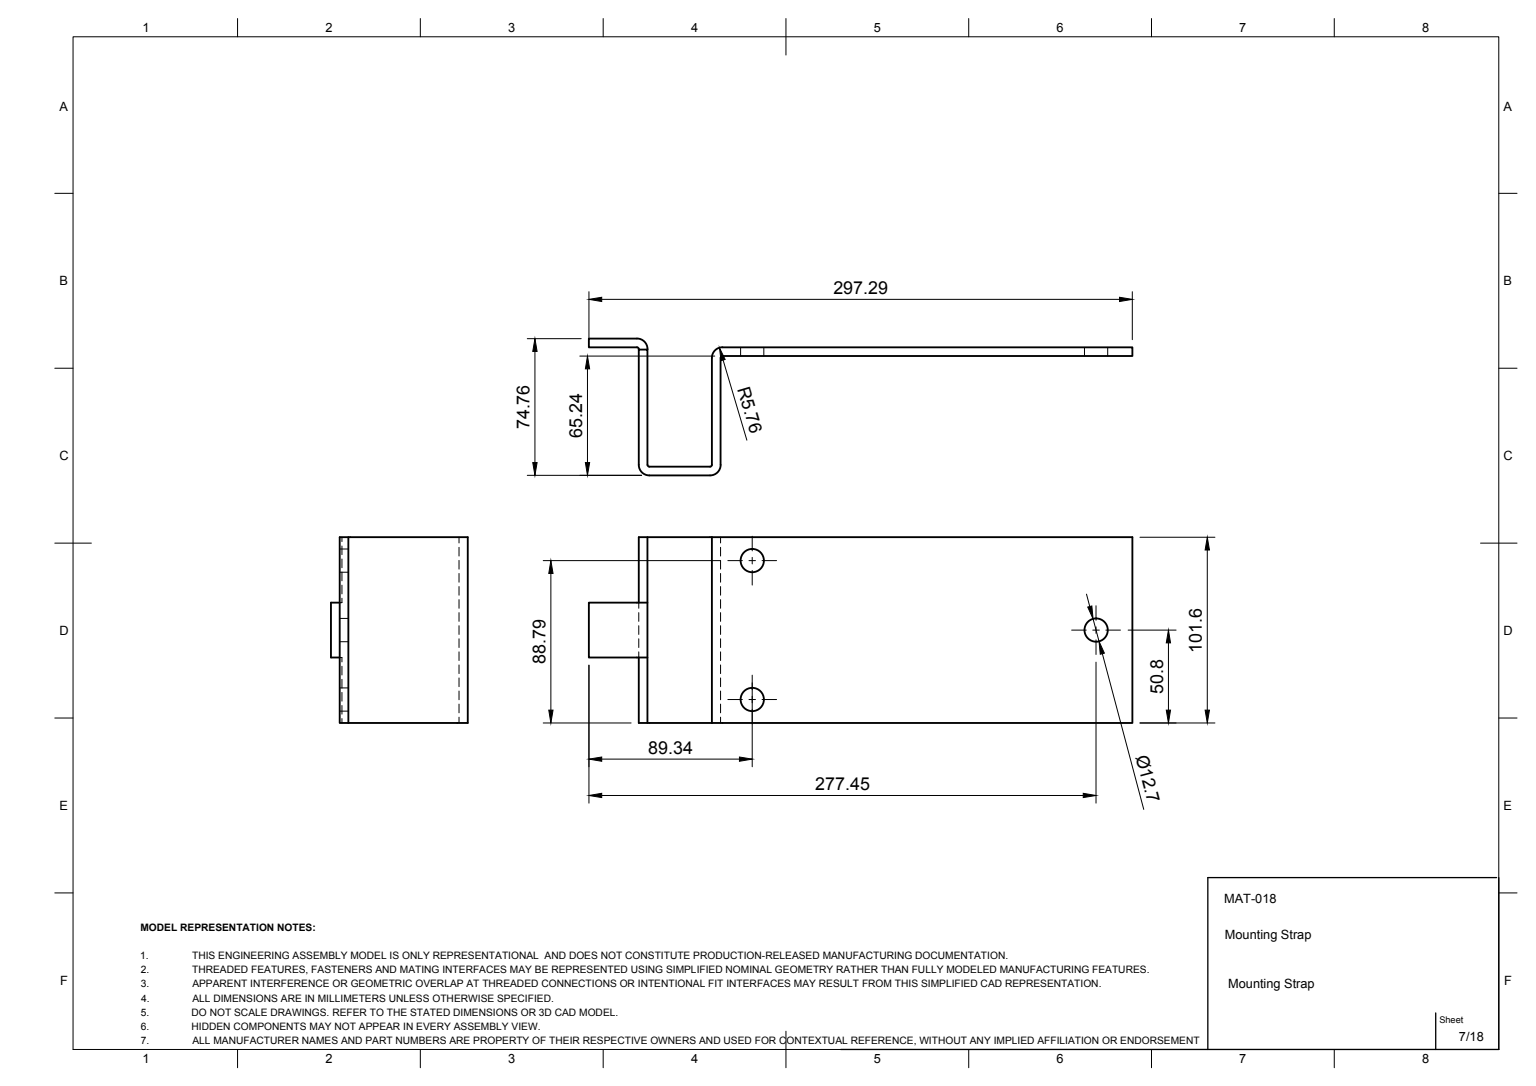
ISO-10303-21;
HEADER;
/* Generated by software containing ST-Developer
 * from STEP Tools, Inc. (www.steptools.com) 
 */

FILE_DESCRIPTION(
/* description */ ('STEP AP214'),
/* implementation_level */ '2;1');

FILE_NAME(
/* name */ 'Mounting Strap.step',
/* time_stamp */ '2026-11-14T06:16:09-08:00',
/* author */ (''),
/* organization */ (''),
/* preprocessor_version */ 'ST-DEVELOPER v20.2',
/* originating_system */ 'Autodesk Translation Framework v15.17.0.0',
/* authorisation */ '');

FILE_SCHEMA (('AUTOMOTIVE_DESIGN { 1 0 10303 214 3 1 1 }'));
ENDSEC;

DATA;
#10=MECHANICAL_DESIGN_GEOMETRIC_PRESENTATION_REPRESENTATION('',(#351),#18006);
#319=SHAPE_REPRESENTATION_RELATIONSHIP('SRR','None',#18075,#335);
#335=ADVANCED_BREP_SHAPE_REPRESENTATION('',(#367),#17992);
#351=STYLED_ITEM('',(#18172),#367);
#367=MANIFOLD_SOLID_BREP('Body1',#9560);
#449=FACE_BOUND('',#1749,.T.);
#450=FACE_BOUND('',#1750,.T.);
#451=FACE_BOUND('',#1751,.T.);
#452=FACE_BOUND('',#1754,.T.);
#453=FACE_BOUND('',#1755,.T.);
#454=FACE_BOUND('',#1756,.T.);
#662=PLANE('',#10157);
#663=PLANE('',#10160);
#664=PLANE('',#10161);
#665=PLANE('',#10164);
#666=PLANE('',#10165);
#667=PLANE('',#10168);
#668=PLANE('',#10169);
#669=PLANE('',#10172);
#670=PLANE('',#10173);
#671=PLANE('',#10176);
#672=PLANE('',#10177);
#673=PLANE('',#10180);
#674=PLANE('',#10181);
#675=PLANE('',#10182);
#676=PLANE('',#10183);
#677=PLANE('',#10184);
#678=PLANE('',#10188);
#679=PLANE('',#10190);
#680=PLANE('',#10192);
#681=PLANE('',#10194);
#682=PLANE('',#10195);
#683=PLANE('',#10196);
#684=PLANE('',#10198);
#685=PLANE('',#10200);
#686=PLANE('',#10202);
#687=PLANE('',#10206);
#688=PLANE('',#10207);
#689=PLANE('',#10208);
#690=PLANE('',#10209);
#691=PLANE('',#10210);
#1076=FACE_OUTER_BOUND('',#1722,.T.);
#1077=FACE_OUTER_BOUND('',#1723,.T.);
#1078=FACE_OUTER_BOUND('',#1724,.T.);
#1079=FACE_OUTER_BOUND('',#1725,.T.);
#1080=FACE_OUTER_BOUND('',#1726,.T.);
#1081=FACE_OUTER_BOUND('',#1727,.T.);
#1082=FACE_OUTER_BOUND('',#1728,.T.);
#1083=FACE_OUTER_BOUND('',#1729,.T.);
#1084=FACE_OUTER_BOUND('',#1730,.T.);
#1085=FACE_OUTER_BOUND('',#1731,.T.);
#1086=FACE_OUTER_BOUND('',#1732,.T.);
#1087=FACE_OUTER_BOUND('',#1733,.T.);
#1088=FACE_OUTER_BOUND('',#1734,.T.);
#1089=FACE_OUTER_BOUND('',#1735,.T.);
#1090=FACE_OUTER_BOUND('',#1736,.T.);
#1091=FACE_OUTER_BOUND('',#1737,.T.);
#1092=FACE_OUTER_BOUND('',#1738,.T.);
#1093=FACE_OUTER_BOUND('',#1739,.T.);
#1094=FACE_OUTER_BOUND('',#1740,.T.);
#1095=FACE_OUTER_BOUND('',#1741,.T.);
#1096=FACE_OUTER_BOUND('',#1742,.T.);
#1097=FACE_OUTER_BOUND('',#1743,.T.);
#1098=FACE_OUTER_BOUND('',#1744,.T.);
#1099=FACE_OUTER_BOUND('',#1745,.T.);
#1100=FACE_OUTER_BOUND('',#1746,.T.);
#1101=FACE_OUTER_BOUND('',#1747,.T.);
#1102=FACE_OUTER_BOUND('',#1748,.T.);
#1103=FACE_OUTER_BOUND('',#1752,.T.);
#1104=FACE_OUTER_BOUND('',#1753,.T.);
#1105=FACE_OUTER_BOUND('',#1757,.T.);
#1106=FACE_OUTER_BOUND('',#1758,.T.);
#1107=FACE_OUTER_BOUND('',#1759,.T.);
#1108=FACE_OUTER_BOUND('',#1760,.T.);
#1109=FACE_OUTER_BOUND('',#1761,.T.);
#1110=FACE_OUTER_BOUND('',#1762,.T.);
#1111=FACE_OUTER_BOUND('',#1763,.T.);
#1112=FACE_OUTER_BOUND('',#1764,.T.);
#1113=FACE_OUTER_BOUND('',#1765,.T.);
#1114=FACE_OUTER_BOUND('',#1766,.T.);
#1115=FACE_OUTER_BOUND('',#1767,.T.);
#1116=FACE_OUTER_BOUND('',#1768,.T.);
#1722=EDGE_LOOP('',(#7242,#7243,#7244,#7245));
#1723=EDGE_LOOP('',(#7246,#7247,#7248,#7249));
#1724=EDGE_LOOP('',(#7250,#7251,#7252,#7253));
#1725=EDGE_LOOP('',(#7254,#7255,#7256,#7257));
#1726=EDGE_LOOP('',(#7258,#7259,#7260,#7261));
#1727=EDGE_LOOP('',(#7262,#7263,#7264,#7265));
#1728=EDGE_LOOP('',(#7266,#7267,#7268,#7269));
#1729=EDGE_LOOP('',(#7270,#7271,#7272,#7273));
#1730=EDGE_LOOP('',(#7274,#7275,#7276,#7277));
#1731=EDGE_LOOP('',(#7278,#7279,#7280,#7281));
#1732=EDGE_LOOP('',(#7282,#7283,#7284,#7285));
#1733=EDGE_LOOP('',(#7286,#7287,#7288,#7289));
#1734=EDGE_LOOP('',(#7290,#7291,#7292,#7293));
#1735=EDGE_LOOP('',(#7294,#7295,#7296,#7297));
#1736=EDGE_LOOP('',(#7298,#7299,#7300,#7301));
#1737=EDGE_LOOP('',(#7302,#7303,#7304,#7305));
#1738=EDGE_LOOP('',(#7306,#7307,#7308,#7309));
#1739=EDGE_LOOP('',(#7310,#7311,#7312,#7313));
#1740=EDGE_LOOP('',(#7314,#7315,#7316,#7317));
#1741=EDGE_LOOP('',(#7318,#7319,#7320,#7321));
#1742=EDGE_LOOP('',(#7322,#7323,#7324,#7325,#7326,#7327,#7328,#7329));
#1743=EDGE_LOOP('',(#7330,#7331,#7332,#7333));
#1744=EDGE_LOOP('',(#7334,#7335,#7336,#7337));
#1745=EDGE_LOOP('',(#7338,#7339,#7340,#7341));
#1746=EDGE_LOOP('',(#7342,#7343,#7344,#7345));
#1747=EDGE_LOOP('',(#7346,#7347,#7348,#7349));
#1748=EDGE_LOOP('',(#7350,#7351,#7352,#7353));
#1749=EDGE_LOOP('',(#7354));
#1750=EDGE_LOOP('',(#7355));
#1751=EDGE_LOOP('',(#7356));
#1752=EDGE_LOOP('',(#7357,#7358,#7359,#7360));
#1753=EDGE_LOOP('',(#7361,#7362,#7363,#7364));
#1754=EDGE_LOOP('',(#7365));
#1755=EDGE_LOOP('',(#7366));
#1756=EDGE_LOOP('',(#7367));
#1757=EDGE_LOOP('',(#7368,#7369,#7370,#7371));
#1758=EDGE_LOOP('',(#7372,#7373,#7374,#7375));
#1759=EDGE_LOOP('',(#7376,#7377,#7378,#7379));
#1760=EDGE_LOOP('',(#7380,#7381,#7382,#7383));
#1761=EDGE_LOOP('',(#7384,#7385,#7386,#7387));
#1762=EDGE_LOOP('',(#7388,#7389,#7390,#7391,#7392,#7393,#7394,#7395));
#1763=EDGE_LOOP('',(#7396,#7397,#7398,#7399));
#1764=EDGE_LOOP('',(#7400,#7401,#7402,#7403));
#1765=EDGE_LOOP('',(#7404,#7405,#7406,#7407,#7408,#7409,#7410,#7411));
#1766=EDGE_LOOP('',(#7412,#7413,#7414,#7415));
#1767=EDGE_LOOP('',(#7416,#7417,#7418,#7419,#7420,#7421,#7422,#7423));
#1768=EDGE_LOOP('',(#7424,#7425,#7426,#7427));
#2503=LINE('',#14917,#3227);
#2504=LINE('',#14923,#3228);
#2505=LINE('',#14929,#3229);
#2506=LINE('',#14934,#3230);
#2507=LINE('',#14938,#3231);
#2508=LINE('',#14942,#3232);
#2509=LINE('',#14944,#3233);
#2510=LINE('',#14945,#3234);
#2511=LINE('',#14949,#3235);
#2512=LINE('',#14953,#3236);
#2513=LINE('',#14957,#3237);
#2514=LINE('',#14959,#3238);
#2515=LINE('',#14960,#3239);
#2516=LINE('',#14964,#3240);
#2517=LINE('',#14969,#3241);
#2518=LINE('',#14971,#3242);
#2519=LINE('',#14972,#3243);
#2520=LINE('',#14976,#3244);
#2521=LINE('',#14980,#3245);
#2522=LINE('',#14983,#3246);
#2523=LINE('',#14984,#3247);
#2524=LINE('',#14988,#3248);
#2525=LINE('',#14994,#3249);
#2526=LINE('',#14995,#3250);
#2527=LINE('',#14996,#3251);
#2528=LINE('',#15000,#3252);
#2529=LINE('',#15004,#3253);
#2530=LINE('',#15007,#3254);
#2531=LINE('',#15008,#3255);
#2532=LINE('',#15012,#3256);
#2533=LINE('',#15013,#3257);
#2534=LINE('',#15014,#3258);
#2535=LINE('',#15018,#3259);
#2536=LINE('',#15020,#3260);
#2537=LINE('',#15022,#3261);
#2538=LINE('',#15023,#3262);
#2539=LINE('',#15026,#3263);
#2540=LINE('',#15028,#3264);
#2541=LINE('',#15029,#3265);
#2542=LINE('',#15032,#3266);
#2543=LINE('',#15034,#3267);
#2544=LINE('',#15035,#3268);
#2545=LINE('',#15041,#3269);
#2546=LINE('',#15044,#3270);
#2547=LINE('',#15046,#3271);
#2548=LINE('',#15047,#3272);
#2549=LINE('',#15048,#3273);
#2550=LINE('',#15049,#3274);
#2551=LINE('',#15051,#3275);
#2552=LINE('',#15053,#3276);
#2553=LINE('',#15055,#3277);
#2554=LINE('',#15057,#3278);
#2555=LINE('',#15059,#3279);
#2556=LINE('',#15062,#3280);
#2557=LINE('',#15063,#3281);
#2558=LINE('',#15066,#3282);
#2559=LINE('',#15067,#3283);
#2560=LINE('',#15069,#3284);
#2561=LINE('',#15070,#3285);
#2562=LINE('',#15072,#3286);
#2563=LINE('',#15074,#3287);
#2564=LINE('',#15076,#3288);
#2565=LINE('',#15078,#3289);
#2566=LINE('',#15080,#3290);
#2567=LINE('',#15084,#3291);
#2568=LINE('',#15086,#3292);
#2569=LINE('',#15087,#3293);
#2570=LINE('',#15089,#3294);
#2571=LINE('',#15090,#3295);
#2572=LINE('',#15096,#3296);
#2573=LINE('',#15099,#3297);
#3227=VECTOR('',#12050,6.34999999999999);
#3228=VECTOR('',#12057,6.34999999999999);
#3229=VECTOR('',#12064,6.35);
#3230=VECTOR('',#12069,1000.);
#3231=VECTOR('',#12072,1000.);
#3232=VECTOR('',#12077,1000.);
#3233=VECTOR('',#12078,1000.);
#3234=VECTOR('',#12079,1000.);
#3235=VECTOR('',#12082,1000.);
#3236=VECTOR('',#12085,1000.);
#3237=VECTOR('',#12090,1000.);
#3238=VECTOR('',#12091,1000.);
#3239=VECTOR('',#12092,1000.);
#3240=VECTOR('',#12095,1000.);
#3241=VECTOR('',#12102,1000.);
#3242=VECTOR('',#12103,1000.);
#3243=VECTOR('',#12104,1000.);
#3244=VECTOR('',#12107,1000.);
#3245=VECTOR('',#12110,1000.);
#3246=VECTOR('',#12115,1000.);
#3247=VECTOR('',#12116,1000.);
#3248=VECTOR('',#12119,1000.);
#3249=VECTOR('',#12126,1000.);
#3250=VECTOR('',#12127,1000.);
#3251=VECTOR('',#12128,1000.);
#3252=VECTOR('',#12131,1000.);
#3253=VECTOR('',#12134,1000.);
#3254=VECTOR('',#12139,1000.);
#3255=VECTOR('',#12140,1000.);
#3256=VECTOR('',#12143,1000.);
#3257=VECTOR('',#12144,1000.);
#3258=VECTOR('',#12145,1000.);
#3259=VECTOR('',#12148,1000.);
#3260=VECTOR('',#12149,1000.);
#3261=VECTOR('',#12150,1000.);
#3262=VECTOR('',#12151,1000.);
#3263=VECTOR('',#12154,1000.);
#3264=VECTOR('',#12155,1000.);
#3265=VECTOR('',#12156,1000.);
#3266=VECTOR('',#12159,1000.);
#3267=VECTOR('',#12160,1000.);
#3268=VECTOR('',#12161,1000.);
#3269=VECTOR('',#12168,1000.);
#3270=VECTOR('',#12171,1000.);
#3271=VECTOR('',#12172,1000.);
#3272=VECTOR('',#12173,1000.);
#3273=VECTOR('',#12174,1000.);
#3274=VECTOR('',#12175,1000.);
#3275=VECTOR('',#12178,1000.);
#3276=VECTOR('',#12181,1000.);
#3277=VECTOR('',#12184,1000.);
#3278=VECTOR('',#12187,1000.);
#3279=VECTOR('',#12190,1000.);
#3280=VECTOR('',#12193,1000.);
#3281=VECTOR('',#12194,1000.);
#3282=VECTOR('',#12197,1000.);
#3283=VECTOR('',#12198,1000.);
#3284=VECTOR('',#12201,1000.);
#3285=VECTOR('',#12202,1000.);
#3286=VECTOR('',#12205,1000.);
#3287=VECTOR('',#12208,1000.);
#3288=VECTOR('',#12211,1000.);
#3289=VECTOR('',#12214,1000.);
#3290=VECTOR('',#12217,1000.);
#3291=VECTOR('',#12220,1000.);
#3292=VECTOR('',#12221,1000.);
#3293=VECTOR('',#12222,1000.);
#3294=VECTOR('',#12223,1000.);
#3295=VECTOR('',#12224,1000.);
#3296=VECTOR('',#12235,1000.);
#3297=VECTOR('',#12240,1000.);
#3714=CIRCLE('',#10149,6.34999999999999);
#3715=CIRCLE('',#10150,6.34999999999999);
#3716=CIRCLE('',#10152,6.34999999999999);
#3717=CIRCLE('',#10153,6.34999999999999);
#3718=CIRCLE('',#10155,6.35);
#3719=CIRCLE('',#10156,6.35);
#3720=CIRCLE('',#10158,1.);
#3721=CIRCLE('',#10159,5.7625);
#3722=CIRCLE('',#10162,1.);
#3723=CIRCLE('',#10163,5.7625);
#3724=CIRCLE('',#10166,5.7625);
#3725=CIRCLE('',#10167,1.);
#3726=CIRCLE('',#10170,5.7625);
#3727=CIRCLE('',#10171,1.);
#3728=CIRCLE('',#10174,5.7625);
#3729=CIRCLE('',#10175,1.);
#3730=CIRCLE('',#10178,5.7625);
#3731=CIRCLE('',#10179,1.);
#3732=CIRCLE('',#10186,1.);
#3733=CIRCLE('',#10187,1.);
#3734=CIRCLE('',#10204,5.7625);
#3735=CIRCLE('',#10205,5.7625);
#4331=VERTEX_POINT('',#14914);
#4332=VERTEX_POINT('',#14916);
#4333=VERTEX_POINT('',#14920);
#4334=VERTEX_POINT('',#14922);
#4335=VERTEX_POINT('',#14926);
#4336=VERTEX_POINT('',#14928);
#4337=VERTEX_POINT('',#14932);
#4338=VERTEX_POINT('',#14933);
#4339=VERTEX_POINT('',#14935);
#4340=VERTEX_POINT('',#14937);
#4341=VERTEX_POINT('',#14941);
#4342=VERTEX_POINT('',#14943);
#4343=VERTEX_POINT('',#14947);
#4344=VERTEX_POINT('',#14948);
#4345=VERTEX_POINT('',#14950);
#4346=VERTEX_POINT('',#14952);
#4347=VERTEX_POINT('',#14956);
#4348=VERTEX_POINT('',#14958);
#4349=VERTEX_POINT('',#14962);
#4350=VERTEX_POINT('',#14963);
#4351=VERTEX_POINT('',#14968);
#4352=VERTEX_POINT('',#14970);
#4353=VERTEX_POINT('',#14974);
#4354=VERTEX_POINT('',#14975);
#4355=VERTEX_POINT('',#14977);
#4356=VERTEX_POINT('',#14979);
#4357=VERTEX_POINT('',#14986);
#4358=VERTEX_POINT('',#14987);
#4359=VERTEX_POINT('',#14992);
#4360=VERTEX_POINT('',#14993);
#4361=VERTEX_POINT('',#14998);
#4362=VERTEX_POINT('',#14999);
#4363=VERTEX_POINT('',#15001);
#4364=VERTEX_POINT('',#15003);
#4365=VERTEX_POINT('',#15010);
#4366=VERTEX_POINT('',#15011);
#4367=VERTEX_POINT('',#15016);
#4368=VERTEX_POINT('',#15017);
#4369=VERTEX_POINT('',#15019);
#4370=VERTEX_POINT('',#15021);
#4371=VERTEX_POINT('',#15025);
#4372=VERTEX_POINT('',#15027);
#4373=VERTEX_POINT('',#15031);
#4374=VERTEX_POINT('',#15033);
#4375=VERTEX_POINT('',#15037);
#4376=VERTEX_POINT('',#15039);
#4377=VERTEX_POINT('',#15043);
#4378=VERTEX_POINT('',#15045);
#4379=VERTEX_POINT('',#15061);
#4380=VERTEX_POINT('',#15065);
#4381=VERTEX_POINT('',#15082);
#4382=VERTEX_POINT('',#15083);
#4383=VERTEX_POINT('',#15085);
#4384=VERTEX_POINT('',#15088);
#5369=EDGE_CURVE('',#4331,#4331,#3714,.T.);
#5370=EDGE_CURVE('',#4331,#4332,#2503,.T.);
#5371=EDGE_CURVE('',#4332,#4332,#3715,.T.);
#5372=EDGE_CURVE('',#4333,#4333,#3716,.T.);
#5373=EDGE_CURVE('',#4333,#4334,#2504,.T.);
#5374=EDGE_CURVE('',#4334,#4334,#3717,.T.);
#5375=EDGE_CURVE('',#4335,#4335,#3718,.T.);
#5376=EDGE_CURVE('',#4335,#4336,#2505,.T.);
#5377=EDGE_CURVE('',#4336,#4336,#3719,.T.);
#5378=EDGE_CURVE('',#4337,#4338,#2506,.T.);
#5379=EDGE_CURVE('',#4339,#4337,#3720,.T.);
#5380=EDGE_CURVE('',#4340,#4339,#2507,.T.);
#5381=EDGE_CURVE('',#4340,#4338,#3721,.T.);
#5382=EDGE_CURVE('',#4337,#4341,#2508,.T.);
#5383=EDGE_CURVE('',#4338,#4342,#2509,.T.);
#5384=EDGE_CURVE('',#4342,#4341,#2510,.T.);
#5385=EDGE_CURVE('',#4343,#4344,#2511,.T.);
#5386=EDGE_CURVE('',#4343,#4345,#3722,.T.);
#5387=EDGE_CURVE('',#4346,#4345,#2512,.T.);
#5388=EDGE_CURVE('',#4344,#4346,#3723,.T.);
#5389=EDGE_CURVE('',#4347,#4343,#2513,.T.);
#5390=EDGE_CURVE('',#4348,#4344,#2514,.T.);
#5391=EDGE_CURVE('',#4348,#4347,#2515,.T.);
#5392=EDGE_CURVE('',#4349,#4350,#2516,.T.);
#5393=EDGE_CURVE('',#4341,#4349,#3724,.T.);
#5394=EDGE_CURVE('',#4342,#4350,#3725,.T.);
#5395=EDGE_CURVE('',#4349,#4351,#2517,.T.);
#5396=EDGE_CURVE('',#4350,#4352,#2518,.T.);
#5397=EDGE_CURVE('',#4352,#4351,#2519,.T.);
#5398=EDGE_CURVE('',#4353,#4354,#2520,.T.);
#5399=EDGE_CURVE('',#4353,#4355,#3726,.T.);
#5400=EDGE_CURVE('',#4356,#4355,#2521,.T.);
#5401=EDGE_CURVE('',#4354,#4356,#3727,.T.);
#5402=EDGE_CURVE('',#4345,#4353,#2522,.T.);
#5403=EDGE_CURVE('',#4346,#4354,#2523,.T.);
#5404=EDGE_CURVE('',#4357,#4358,#2524,.T.);
#5405=EDGE_CURVE('',#4351,#4357,#3728,.T.);
#5406=EDGE_CURVE('',#4352,#4358,#3729,.T.);
#5407=EDGE_CURVE('',#4359,#4360,#2525,.T.);
#5408=EDGE_CURVE('',#4357,#4359,#2526,.T.);
#5409=EDGE_CURVE('',#4358,#4360,#2527,.T.);
#5410=EDGE_CURVE('',#4361,#4362,#2528,.T.);
#5411=EDGE_CURVE('',#4361,#4363,#3730,.T.);
#5412=EDGE_CURVE('',#4364,#4363,#2529,.T.);
#5413=EDGE_CURVE('',#4362,#4364,#3731,.T.);
#5414=EDGE_CURVE('',#4355,#4361,#2530,.T.);
#5415=EDGE_CURVE('',#4356,#4362,#2531,.T.);
#5416=EDGE_CURVE('',#4365,#4366,#2532,.T.);
#5417=EDGE_CURVE('',#4364,#4366,#2533,.T.);
#5418=EDGE_CURVE('',#4363,#4365,#2534,.T.);
#5419=EDGE_CURVE('',#4367,#4368,#2535,.T.);
#5420=EDGE_CURVE('',#4367,#4369,#2536,.T.);
#5421=EDGE_CURVE('',#4369,#4370,#2537,.T.);
#5422=EDGE_CURVE('',#4368,#4370,#2538,.T.);
#5423=EDGE_CURVE('',#4367,#4371,#2539,.T.);
#5424=EDGE_CURVE('',#4372,#4368,#2540,.T.);
#5425=EDGE_CURVE('',#4371,#4372,#2541,.T.);
#5426=EDGE_CURVE('',#4371,#4373,#2542,.T.);
#5427=EDGE_CURVE('',#4374,#4372,#2543,.T.);
#5428=EDGE_CURVE('',#4373,#4374,#2544,.T.);
#5429=EDGE_CURVE('',#4373,#4375,#3732,.T.);
#5430=EDGE_CURVE('',#4376,#4374,#3733,.T.);
#5431=EDGE_CURVE('',#4375,#4376,#2545,.T.);
#5432=EDGE_CURVE('',#4375,#4377,#2546,.T.);
#5433=EDGE_CURVE('',#4378,#4376,#2547,.T.);
#5434=EDGE_CURVE('',#4365,#4378,#2548,.T.);
#5435=EDGE_CURVE('',#4357,#4363,#2549,.T.);
#5436=EDGE_CURVE('',#4377,#4359,#2550,.T.);
#5437=EDGE_CURVE('',#4351,#4361,#2551,.T.);
#5438=EDGE_CURVE('',#4349,#4355,#2552,.T.);
#5439=EDGE_CURVE('',#4341,#4353,#2553,.T.);
#5440=EDGE_CURVE('',#4337,#4345,#2554,.T.);
#5441=EDGE_CURVE('',#4339,#4343,#2555,.T.);
#5442=EDGE_CURVE('',#4379,#4347,#2556,.T.);
#5443=EDGE_CURVE('',#4379,#4339,#2557,.T.);
#5444=EDGE_CURVE('',#4380,#4348,#2558,.T.);
#5445=EDGE_CURVE('',#4380,#4379,#2559,.T.);
#5446=EDGE_CURVE('',#4340,#4344,#2560,.T.);
#5447=EDGE_CURVE('',#4380,#4340,#2561,.T.);
#5448=EDGE_CURVE('',#4338,#4346,#2562,.T.);
#5449=EDGE_CURVE('',#4342,#4354,#2563,.T.);
#5450=EDGE_CURVE('',#4350,#4356,#2564,.T.);
#5451=EDGE_CURVE('',#4352,#4362,#2565,.T.);
#5452=EDGE_CURVE('',#4358,#4364,#2566,.T.);
#5453=EDGE_CURVE('',#4381,#4382,#2567,.T.);
#5454=EDGE_CURVE('',#4383,#4381,#2568,.T.);
#5455=EDGE_CURVE('',#4360,#4383,#2569,.T.);
#5456=EDGE_CURVE('',#4384,#4366,#2570,.T.);
#5457=EDGE_CURVE('',#4382,#4384,#2571,.T.);
#5458=EDGE_CURVE('',#4369,#4381,#3734,.T.);
#5459=EDGE_CURVE('',#4382,#4370,#3735,.T.);
#5460=EDGE_CURVE('',#4378,#4384,#2572,.T.);
#5461=EDGE_CURVE('',#4377,#4383,#2573,.T.);
#7242=ORIENTED_EDGE('',*,*,#5369,.F.);
#7243=ORIENTED_EDGE('',*,*,#5370,.T.);
#7244=ORIENTED_EDGE('',*,*,#5371,.T.);
#7245=ORIENTED_EDGE('',*,*,#5370,.F.);
#7246=ORIENTED_EDGE('',*,*,#5372,.F.);
#7247=ORIENTED_EDGE('',*,*,#5373,.T.);
#7248=ORIENTED_EDGE('',*,*,#5374,.T.);
#7249=ORIENTED_EDGE('',*,*,#5373,.F.);
#7250=ORIENTED_EDGE('',*,*,#5375,.F.);
#7251=ORIENTED_EDGE('',*,*,#5376,.T.);
#7252=ORIENTED_EDGE('',*,*,#5377,.T.);
#7253=ORIENTED_EDGE('',*,*,#5376,.F.);
#7254=ORIENTED_EDGE('',*,*,#5378,.F.);
#7255=ORIENTED_EDGE('',*,*,#5379,.F.);
#7256=ORIENTED_EDGE('',*,*,#5380,.F.);
#7257=ORIENTED_EDGE('',*,*,#5381,.T.);
#7258=ORIENTED_EDGE('',*,*,#5382,.F.);
#7259=ORIENTED_EDGE('',*,*,#5378,.T.);
#7260=ORIENTED_EDGE('',*,*,#5383,.T.);
#7261=ORIENTED_EDGE('',*,*,#5384,.T.);
#7262=ORIENTED_EDGE('',*,*,#5385,.F.);
#7263=ORIENTED_EDGE('',*,*,#5386,.T.);
#7264=ORIENTED_EDGE('',*,*,#5387,.F.);
#7265=ORIENTED_EDGE('',*,*,#5388,.F.);
#7266=ORIENTED_EDGE('',*,*,#5389,.T.);
#7267=ORIENTED_EDGE('',*,*,#5385,.T.);
#7268=ORIENTED_EDGE('',*,*,#5390,.F.);
#7269=ORIENTED_EDGE('',*,*,#5391,.T.);
#7270=ORIENTED_EDGE('',*,*,#5392,.F.);
#7271=ORIENTED_EDGE('',*,*,#5393,.F.);
#7272=ORIENTED_EDGE('',*,*,#5384,.F.);
#7273=ORIENTED_EDGE('',*,*,#5394,.T.);
#7274=ORIENTED_EDGE('',*,*,#5395,.F.);
#7275=ORIENTED_EDGE('',*,*,#5392,.T.);
#7276=ORIENTED_EDGE('',*,*,#5396,.T.);
#7277=ORIENTED_EDGE('',*,*,#5397,.T.);
#7278=ORIENTED_EDGE('',*,*,#5398,.F.);
#7279=ORIENTED_EDGE('',*,*,#5399,.T.);
#7280=ORIENTED_EDGE('',*,*,#5400,.F.);
#7281=ORIENTED_EDGE('',*,*,#5401,.F.);
#7282=ORIENTED_EDGE('',*,*,#5402,.T.);
#7283=ORIENTED_EDGE('',*,*,#5398,.T.);
#7284=ORIENTED_EDGE('',*,*,#5403,.F.);
#7285=ORIENTED_EDGE('',*,*,#5387,.T.);
#7286=ORIENTED_EDGE('',*,*,#5404,.F.);
#7287=ORIENTED_EDGE('',*,*,#5405,.F.);
#7288=ORIENTED_EDGE('',*,*,#5397,.F.);
#7289=ORIENTED_EDGE('',*,*,#5406,.T.);
#7290=ORIENTED_EDGE('',*,*,#5407,.F.);
#7291=ORIENTED_EDGE('',*,*,#5408,.F.);
#7292=ORIENTED_EDGE('',*,*,#5404,.T.);
#7293=ORIENTED_EDGE('',*,*,#5409,.T.);
#7294=ORIENTED_EDGE('',*,*,#5410,.F.);
#7295=ORIENTED_EDGE('',*,*,#5411,.T.);
#7296=ORIENTED_EDGE('',*,*,#5412,.F.);
#7297=ORIENTED_EDGE('',*,*,#5413,.F.);
#7298=ORIENTED_EDGE('',*,*,#5414,.T.);
#7299=ORIENTED_EDGE('',*,*,#5410,.T.);
#7300=ORIENTED_EDGE('',*,*,#5415,.F.);
#7301=ORIENTED_EDGE('',*,*,#5400,.T.);
#7302=ORIENTED_EDGE('',*,*,#5416,.T.);
#7303=ORIENTED_EDGE('',*,*,#5417,.F.);
#7304=ORIENTED_EDGE('',*,*,#5412,.T.);
#7305=ORIENTED_EDGE('',*,*,#5418,.T.);
#7306=ORIENTED_EDGE('',*,*,#5419,.F.);
#7307=ORIENTED_EDGE('',*,*,#5420,.T.);
#7308=ORIENTED_EDGE('',*,*,#5421,.T.);
#7309=ORIENTED_EDGE('',*,*,#5422,.F.);
#7310=ORIENTED_EDGE('',*,*,#5423,.F.);
#7311=ORIENTED_EDGE('',*,*,#5419,.T.);
#7312=ORIENTED_EDGE('',*,*,#5424,.F.);
#7313=ORIENTED_EDGE('',*,*,#5425,.F.);
#7314=ORIENTED_EDGE('',*,*,#5426,.F.);
#7315=ORIENTED_EDGE('',*,*,#5425,.T.);
#7316=ORIENTED_EDGE('',*,*,#5427,.F.);
#7317=ORIENTED_EDGE('',*,*,#5428,.F.);
#7318=ORIENTED_EDGE('',*,*,#5429,.F.);
#7319=ORIENTED_EDGE('',*,*,#5428,.T.);
#7320=ORIENTED_EDGE('',*,*,#5430,.F.);
#7321=ORIENTED_EDGE('',*,*,#5431,.F.);
#7322=ORIENTED_EDGE('',*,*,#5432,.F.);
#7323=ORIENTED_EDGE('',*,*,#5431,.T.);
#7324=ORIENTED_EDGE('',*,*,#5433,.F.);
#7325=ORIENTED_EDGE('',*,*,#5434,.F.);
#7326=ORIENTED_EDGE('',*,*,#5418,.F.);
#7327=ORIENTED_EDGE('',*,*,#5435,.F.);
#7328=ORIENTED_EDGE('',*,*,#5408,.T.);
#7329=ORIENTED_EDGE('',*,*,#5436,.F.);
#7330=ORIENTED_EDGE('',*,*,#5411,.F.);
#7331=ORIENTED_EDGE('',*,*,#5437,.F.);
#7332=ORIENTED_EDGE('',*,*,#5405,.T.);
#7333=ORIENTED_EDGE('',*,*,#5435,.T.);
#7334=ORIENTED_EDGE('',*,*,#5414,.F.);
#7335=ORIENTED_EDGE('',*,*,#5438,.F.);
#7336=ORIENTED_EDGE('',*,*,#5395,.T.);
#7337=ORIENTED_EDGE('',*,*,#5437,.T.);
#7338=ORIENTED_EDGE('',*,*,#5399,.F.);
#7339=ORIENTED_EDGE('',*,*,#5439,.F.);
#7340=ORIENTED_EDGE('',*,*,#5393,.T.);
#7341=ORIENTED_EDGE('',*,*,#5438,.T.);
#7342=ORIENTED_EDGE('',*,*,#5402,.F.);
#7343=ORIENTED_EDGE('',*,*,#5440,.F.);
#7344=ORIENTED_EDGE('',*,*,#5382,.T.);
#7345=ORIENTED_EDGE('',*,*,#5439,.T.);
#7346=ORIENTED_EDGE('',*,*,#5386,.F.);
#7347=ORIENTED_EDGE('',*,*,#5441,.F.);
#7348=ORIENTED_EDGE('',*,*,#5379,.T.);
#7349=ORIENTED_EDGE('',*,*,#5440,.T.);
#7350=ORIENTED_EDGE('',*,*,#5389,.F.);
#7351=ORIENTED_EDGE('',*,*,#5442,.F.);
#7352=ORIENTED_EDGE('',*,*,#5443,.T.);
#7353=ORIENTED_EDGE('',*,*,#5441,.T.);
#7354=ORIENTED_EDGE('',*,*,#5371,.F.);
#7355=ORIENTED_EDGE('',*,*,#5374,.F.);
#7356=ORIENTED_EDGE('',*,*,#5377,.F.);
#7357=ORIENTED_EDGE('',*,*,#5391,.F.);
#7358=ORIENTED_EDGE('',*,*,#5444,.F.);
#7359=ORIENTED_EDGE('',*,*,#5445,.T.);
#7360=ORIENTED_EDGE('',*,*,#5442,.T.);
#7361=ORIENTED_EDGE('',*,*,#5390,.T.);
#7362=ORIENTED_EDGE('',*,*,#5446,.F.);
#7363=ORIENTED_EDGE('',*,*,#5447,.F.);
#7364=ORIENTED_EDGE('',*,*,#5444,.T.);
#7365=ORIENTED_EDGE('',*,*,#5369,.T.);
#7366=ORIENTED_EDGE('',*,*,#5372,.T.);
#7367=ORIENTED_EDGE('',*,*,#5375,.T.);
#7368=ORIENTED_EDGE('',*,*,#5388,.T.);
#7369=ORIENTED_EDGE('',*,*,#5448,.F.);
#7370=ORIENTED_EDGE('',*,*,#5381,.F.);
#7371=ORIENTED_EDGE('',*,*,#5446,.T.);
#7372=ORIENTED_EDGE('',*,*,#5403,.T.);
#7373=ORIENTED_EDGE('',*,*,#5449,.F.);
#7374=ORIENTED_EDGE('',*,*,#5383,.F.);
#7375=ORIENTED_EDGE('',*,*,#5448,.T.);
#7376=ORIENTED_EDGE('',*,*,#5401,.T.);
#7377=ORIENTED_EDGE('',*,*,#5450,.F.);
#7378=ORIENTED_EDGE('',*,*,#5394,.F.);
#7379=ORIENTED_EDGE('',*,*,#5449,.T.);
#7380=ORIENTED_EDGE('',*,*,#5415,.T.);
#7381=ORIENTED_EDGE('',*,*,#5451,.F.);
#7382=ORIENTED_EDGE('',*,*,#5396,.F.);
#7383=ORIENTED_EDGE('',*,*,#5450,.T.);
#7384=ORIENTED_EDGE('',*,*,#5413,.T.);
#7385=ORIENTED_EDGE('',*,*,#5452,.F.);
#7386=ORIENTED_EDGE('',*,*,#5406,.F.);
#7387=ORIENTED_EDGE('',*,*,#5451,.T.);
#7388=ORIENTED_EDGE('',*,*,#5453,.F.);
#7389=ORIENTED_EDGE('',*,*,#5454,.F.);
#7390=ORIENTED_EDGE('',*,*,#5455,.F.);
#7391=ORIENTED_EDGE('',*,*,#5409,.F.);
#7392=ORIENTED_EDGE('',*,*,#5452,.T.);
#7393=ORIENTED_EDGE('',*,*,#5417,.T.);
#7394=ORIENTED_EDGE('',*,*,#5456,.F.);
#7395=ORIENTED_EDGE('',*,*,#5457,.F.);
#7396=ORIENTED_EDGE('',*,*,#5421,.F.);
#7397=ORIENTED_EDGE('',*,*,#5458,.T.);
#7398=ORIENTED_EDGE('',*,*,#5453,.T.);
#7399=ORIENTED_EDGE('',*,*,#5459,.T.);
#7400=ORIENTED_EDGE('',*,*,#5447,.T.);
#7401=ORIENTED_EDGE('',*,*,#5380,.T.);
#7402=ORIENTED_EDGE('',*,*,#5443,.F.);
#7403=ORIENTED_EDGE('',*,*,#5445,.F.);
#7404=ORIENTED_EDGE('',*,*,#5424,.T.);
#7405=ORIENTED_EDGE('',*,*,#5422,.T.);
#7406=ORIENTED_EDGE('',*,*,#5459,.F.);
#7407=ORIENTED_EDGE('',*,*,#5457,.T.);
#7408=ORIENTED_EDGE('',*,*,#5460,.F.);
#7409=ORIENTED_EDGE('',*,*,#5433,.T.);
#7410=ORIENTED_EDGE('',*,*,#5430,.T.);
#7411=ORIENTED_EDGE('',*,*,#5427,.T.);
#7412=ORIENTED_EDGE('',*,*,#5434,.T.);
#7413=ORIENTED_EDGE('',*,*,#5460,.T.);
#7414=ORIENTED_EDGE('',*,*,#5456,.T.);
#7415=ORIENTED_EDGE('',*,*,#5416,.F.);
#7416=ORIENTED_EDGE('',*,*,#5423,.T.);
#7417=ORIENTED_EDGE('',*,*,#5426,.T.);
#7418=ORIENTED_EDGE('',*,*,#5429,.T.);
#7419=ORIENTED_EDGE('',*,*,#5432,.T.);
#7420=ORIENTED_EDGE('',*,*,#5461,.T.);
#7421=ORIENTED_EDGE('',*,*,#5454,.T.);
#7422=ORIENTED_EDGE('',*,*,#5458,.F.);
#7423=ORIENTED_EDGE('',*,*,#5420,.F.);
#7424=ORIENTED_EDGE('',*,*,#5436,.T.);
#7425=ORIENTED_EDGE('',*,*,#5407,.T.);
#7426=ORIENTED_EDGE('',*,*,#5455,.T.);
#7427=ORIENTED_EDGE('',*,*,#5461,.F.);
#8883=CYLINDRICAL_SURFACE('',#10148,6.34999999999999);
#8884=CYLINDRICAL_SURFACE('',#10151,6.34999999999999);
#8885=CYLINDRICAL_SURFACE('',#10154,6.35);
#8886=CYLINDRICAL_SURFACE('',#10185,1.);
#8887=CYLINDRICAL_SURFACE('',#10189,5.7625);
#8888=CYLINDRICAL_SURFACE('',#10191,5.7625);
#8889=CYLINDRICAL_SURFACE('',#10193,1.);
#8890=CYLINDRICAL_SURFACE('',#10197,5.7625);
#8891=CYLINDRICAL_SURFACE('',#10199,1.);
#8892=CYLINDRICAL_SURFACE('',#10201,1.);
#8893=CYLINDRICAL_SURFACE('',#10203,5.7625);
#9215=ADVANCED_FACE('',(#1076),#8883,.F.);
#9216=ADVANCED_FACE('',(#1077),#8884,.F.);
#9217=ADVANCED_FACE('',(#1078),#8885,.F.);
#9218=ADVANCED_FACE('',(#1079),#662,.T.);
#9219=ADVANCED_FACE('',(#1080),#663,.T.);
#9220=ADVANCED_FACE('',(#1081),#664,.T.);
#9221=ADVANCED_FACE('',(#1082),#665,.T.);
#9222=ADVANCED_FACE('',(#1083),#666,.T.);
#9223=ADVANCED_FACE('',(#1084),#667,.T.);
#9224=ADVANCED_FACE('',(#1085),#668,.T.);
#9225=ADVANCED_FACE('',(#1086),#669,.T.);
#9226=ADVANCED_FACE('',(#1087),#670,.T.);
#9227=ADVANCED_FACE('',(#1088),#671,.T.);
#9228=ADVANCED_FACE('',(#1089),#672,.T.);
#9229=ADVANCED_FACE('',(#1090),#673,.T.);
#9230=ADVANCED_FACE('',(#1091),#674,.T.);
#9231=ADVANCED_FACE('',(#1092),#675,.F.);
#9232=ADVANCED_FACE('',(#1093),#676,.T.);
#9233=ADVANCED_FACE('',(#1094),#677,.T.);
#9234=ADVANCED_FACE('',(#1095),#8886,.F.);
#9235=ADVANCED_FACE('',(#1096),#678,.T.);
#9236=ADVANCED_FACE('',(#1097),#8887,.T.);
#9237=ADVANCED_FACE('',(#1098),#679,.T.);
#9238=ADVANCED_FACE('',(#1099),#8888,.T.);
#9239=ADVANCED_FACE('',(#1100),#680,.T.);
#9240=ADVANCED_FACE('',(#1101),#8889,.F.);
#9241=ADVANCED_FACE('',(#1102,#449,#450,#451),#681,.T.);
#9242=ADVANCED_FACE('',(#1103),#682,.T.);
#9243=ADVANCED_FACE('',(#1104,#452,#453,#454),#683,.F.);
#9244=ADVANCED_FACE('',(#1105),#8890,.T.);
#9245=ADVANCED_FACE('',(#1106),#684,.F.);
#9246=ADVANCED_FACE('',(#1107),#8891,.F.);
#9247=ADVANCED_FACE('',(#1108),#685,.F.);
#9248=ADVANCED_FACE('',(#1109),#8892,.F.);
#9249=ADVANCED_FACE('',(#1110),#686,.F.);
#9250=ADVANCED_FACE('',(#1111),#8893,.T.);
#9251=ADVANCED_FACE('',(#1112),#687,.F.);
#9252=ADVANCED_FACE('',(#1113),#688,.F.);
#9253=ADVANCED_FACE('',(#1114),#689,.F.);
#9254=ADVANCED_FACE('',(#1115),#690,.F.);
#9255=ADVANCED_FACE('',(#1116),#691,.F.);
#9560=CLOSED_SHELL('',(#9215,#9216,#9217,#9218,#9219,#9220,#9221,#9222,
#9223,#9224,#9225,#9226,#9227,#9228,#9229,#9230,#9231,#9232,#9233,#9234,
#9235,#9236,#9237,#9238,#9239,#9240,#9241,#9242,#9243,#9244,#9245,#9246,
#9247,#9248,#9249,#9250,#9251,#9252,#9253,#9254,#9255));
#10147=AXIS2_PLACEMENT_3D('',#14912,#12044,#12045);
#10148=AXIS2_PLACEMENT_3D('',#14913,#12046,#12047);
#10149=AXIS2_PLACEMENT_3D('',#14915,#12048,#12049);
#10150=AXIS2_PLACEMENT_3D('',#14918,#12051,#12052);
#10151=AXIS2_PLACEMENT_3D('',#14919,#12053,#12054);
#10152=AXIS2_PLACEMENT_3D('',#14921,#12055,#12056);
#10153=AXIS2_PLACEMENT_3D('',#14924,#12058,#12059);
#10154=AXIS2_PLACEMENT_3D('',#14925,#12060,#12061);
#10155=AXIS2_PLACEMENT_3D('',#14927,#12062,#12063);
#10156=AXIS2_PLACEMENT_3D('',#14930,#12065,#12066);
#10157=AXIS2_PLACEMENT_3D('',#14931,#12067,#12068);
#10158=AXIS2_PLACEMENT_3D('',#14936,#12070,#12071);
#10159=AXIS2_PLACEMENT_3D('',#14939,#12073,#12074);
#10160=AXIS2_PLACEMENT_3D('',#14940,#12075,#12076);
#10161=AXIS2_PLACEMENT_3D('',#14946,#12080,#12081);
#10162=AXIS2_PLACEMENT_3D('',#14951,#12083,#12084);
#10163=AXIS2_PLACEMENT_3D('',#14954,#12086,#12087);
#10164=AXIS2_PLACEMENT_3D('',#14955,#12088,#12089);
#10165=AXIS2_PLACEMENT_3D('',#14961,#12093,#12094);
#10166=AXIS2_PLACEMENT_3D('',#14965,#12096,#12097);
#10167=AXIS2_PLACEMENT_3D('',#14966,#12098,#12099);
#10168=AXIS2_PLACEMENT_3D('',#14967,#12100,#12101);
#10169=AXIS2_PLACEMENT_3D('',#14973,#12105,#12106);
#10170=AXIS2_PLACEMENT_3D('',#14978,#12108,#12109);
#10171=AXIS2_PLACEMENT_3D('',#14981,#12111,#12112);
#10172=AXIS2_PLACEMENT_3D('',#14982,#12113,#12114);
#10173=AXIS2_PLACEMENT_3D('',#14985,#12117,#12118);
#10174=AXIS2_PLACEMENT_3D('',#14989,#12120,#12121);
#10175=AXIS2_PLACEMENT_3D('',#14990,#12122,#12123);
#10176=AXIS2_PLACEMENT_3D('',#14991,#12124,#12125);
#10177=AXIS2_PLACEMENT_3D('',#14997,#12129,#12130);
#10178=AXIS2_PLACEMENT_3D('',#15002,#12132,#12133);
#10179=AXIS2_PLACEMENT_3D('',#15005,#12135,#12136);
#10180=AXIS2_PLACEMENT_3D('',#15006,#12137,#12138);
#10181=AXIS2_PLACEMENT_3D('',#15009,#12141,#12142);
#10182=AXIS2_PLACEMENT_3D('',#15015,#12146,#12147);
#10183=AXIS2_PLACEMENT_3D('',#15024,#12152,#12153);
#10184=AXIS2_PLACEMENT_3D('',#15030,#12157,#12158);
#10185=AXIS2_PLACEMENT_3D('',#15036,#12162,#12163);
#10186=AXIS2_PLACEMENT_3D('',#15038,#12164,#12165);
#10187=AXIS2_PLACEMENT_3D('',#15040,#12166,#12167);
#10188=AXIS2_PLACEMENT_3D('',#15042,#12169,#12170);
#10189=AXIS2_PLACEMENT_3D('',#15050,#12176,#12177);
#10190=AXIS2_PLACEMENT_3D('',#15052,#12179,#12180);
#10191=AXIS2_PLACEMENT_3D('',#15054,#12182,#12183);
#10192=AXIS2_PLACEMENT_3D('',#15056,#12185,#12186);
#10193=AXIS2_PLACEMENT_3D('',#15058,#12188,#12189);
#10194=AXIS2_PLACEMENT_3D('',#15060,#12191,#12192);
#10195=AXIS2_PLACEMENT_3D('',#15064,#12195,#12196);
#10196=AXIS2_PLACEMENT_3D('',#15068,#12199,#12200);
#10197=AXIS2_PLACEMENT_3D('',#15071,#12203,#12204);
#10198=AXIS2_PLACEMENT_3D('',#15073,#12206,#12207);
#10199=AXIS2_PLACEMENT_3D('',#15075,#12209,#12210);
#10200=AXIS2_PLACEMENT_3D('',#15077,#12212,#12213);
#10201=AXIS2_PLACEMENT_3D('',#15079,#12215,#12216);
#10202=AXIS2_PLACEMENT_3D('',#15081,#12218,#12219);
#10203=AXIS2_PLACEMENT_3D('',#15091,#12225,#12226);
#10204=AXIS2_PLACEMENT_3D('',#15092,#12227,#12228);
#10205=AXIS2_PLACEMENT_3D('',#15093,#12229,#12230);
#10206=AXIS2_PLACEMENT_3D('',#15094,#12231,#12232);
#10207=AXIS2_PLACEMENT_3D('',#15095,#12233,#12234);
#10208=AXIS2_PLACEMENT_3D('',#15097,#12236,#12237);
#10209=AXIS2_PLACEMENT_3D('',#15098,#12238,#12239);
#10210=AXIS2_PLACEMENT_3D('',#15100,#12241,#12242);
#12044=DIRECTION('axis',(0.,0.,1.));
#12045=DIRECTION('refdir',(1.,0.,0.));
#12046=DIRECTION('center_axis',(0.,1.,0.));
#12047=DIRECTION('ref_axis',(0.,0.,1.));
#12048=DIRECTION('center_axis',(0.,1.,0.));
#12049=DIRECTION('ref_axis',(0.,0.,1.));
#12050=DIRECTION('',(0.,1.,0.));
#12051=DIRECTION('center_axis',(0.,1.,0.));
#12052=DIRECTION('ref_axis',(0.,0.,1.));
#12053=DIRECTION('center_axis',(0.,1.,0.));
#12054=DIRECTION('ref_axis',(0.,0.,1.));
#12055=DIRECTION('center_axis',(0.,1.,0.));
#12056=DIRECTION('ref_axis',(0.,0.,1.));
#12057=DIRECTION('',(0.,1.,0.));
#12058=DIRECTION('center_axis',(0.,1.,0.));
#12059=DIRECTION('ref_axis',(0.,0.,-1.));
#12060=DIRECTION('center_axis',(0.,1.,0.));
#12061=DIRECTION('ref_axis',(0.,0.,1.));
#12062=DIRECTION('center_axis',(0.,1.,0.));
#12063=DIRECTION('ref_axis',(0.,0.,1.));
#12064=DIRECTION('',(0.,1.,0.));
#12065=DIRECTION('center_axis',(0.,1.,0.));
#12066=DIRECTION('ref_axis',(0.,0.,1.));
#12067=DIRECTION('center_axis',(0.,0.,1.));
#12068=DIRECTION('ref_axis',(1.,0.,0.));
#12069=DIRECTION('',(1.,-9.10615997888087E-17,0.));
#12070=DIRECTION('center_axis',(0.,0.,1.));
#12071=DIRECTION('ref_axis',(-1.,0.,0.));
#12072=DIRECTION('',(0.,1.,0.));
#12073=DIRECTION('center_axis',(0.,0.,1.));
#12074=DIRECTION('ref_axis',(1.,0.,0.));
#12075=DIRECTION('center_axis',(0.,0.,1.));
#12076=DIRECTION('ref_axis',(1.,0.,0.));
#12077=DIRECTION('',(0.,1.,0.));
#12078=DIRECTION('',(0.,1.,0.));
#12079=DIRECTION('',(-1.,0.,0.));
#12080=DIRECTION('center_axis',(0.,0.,-1.));
#12081=DIRECTION('ref_axis',(-1.,0.,0.));
#12082=DIRECTION('',(0.,-1.,0.));
#12083=DIRECTION('center_axis',(0.,0.,1.));
#12084=DIRECTION('ref_axis',(-1.,0.,0.));
#12085=DIRECTION('',(-1.,9.10615997888087E-17,0.));
#12086=DIRECTION('center_axis',(0.,0.,1.));
#12087=DIRECTION('ref_axis',(1.,0.,0.));
#12088=DIRECTION('center_axis',(0.,0.,-1.));
#12089=DIRECTION('ref_axis',(-1.,0.,0.));
#12090=DIRECTION('',(1.,0.,0.));
#12091=DIRECTION('',(1.,0.,0.));
#12092=DIRECTION('',(0.,1.,0.));
#12093=DIRECTION('center_axis',(0.,0.,1.));
#12094=DIRECTION('ref_axis',(1.,0.,0.));
#12095=DIRECTION('',(0.,-1.,0.));
#12096=DIRECTION('center_axis',(0.,0.,-1.));
#12097=DIRECTION('ref_axis',(1.,0.,0.));
#12098=DIRECTION('center_axis',(0.,0.,-1.));
#12099=DIRECTION('ref_axis',(1.,0.,0.));
#12100=DIRECTION('center_axis',(0.,0.,1.));
#12101=DIRECTION('ref_axis',(1.,0.,0.));
#12102=DIRECTION('',(1.,0.,0.));
#12103=DIRECTION('',(1.,0.,0.));
#12104=DIRECTION('',(0.,1.,0.));
#12105=DIRECTION('center_axis',(0.,0.,-1.));
#12106=DIRECTION('ref_axis',(-1.,0.,0.));
#12107=DIRECTION('',(1.,0.,0.));
#12108=DIRECTION('center_axis',(0.,0.,-1.));
#12109=DIRECTION('ref_axis',(1.,0.,0.));
#12110=DIRECTION('',(0.,1.,0.));
#12111=DIRECTION('center_axis',(0.,0.,-1.));
#12112=DIRECTION('ref_axis',(1.,0.,0.));
#12113=DIRECTION('center_axis',(0.,0.,-1.));
#12114=DIRECTION('ref_axis',(-1.,0.,0.));
#12115=DIRECTION('',(0.,1.,0.));
#12116=DIRECTION('',(0.,1.,0.));
#12117=DIRECTION('center_axis',(0.,0.,1.));
#12118=DIRECTION('ref_axis',(1.,0.,0.));
#12119=DIRECTION('',(-1.,0.,0.));
#12120=DIRECTION('center_axis',(0.,0.,-1.));
#12121=DIRECTION('ref_axis',(1.,0.,0.));
#12122=DIRECTION('center_axis',(0.,0.,-1.));
#12123=DIRECTION('ref_axis',(1.,0.,0.));
#12124=DIRECTION('center_axis',(0.,0.,1.));
#12125=DIRECTION('ref_axis',(1.,0.,0.));
#12126=DIRECTION('',(-1.,0.,0.));
#12127=DIRECTION('',(0.,-1.,0.));
#12128=DIRECTION('',(0.,-1.,0.));
#12129=DIRECTION('center_axis',(0.,0.,-1.));
#12130=DIRECTION('ref_axis',(-1.,0.,0.));
#12131=DIRECTION('',(0.,-1.,0.));
#12132=DIRECTION('center_axis',(0.,0.,-1.));
#12133=DIRECTION('ref_axis',(1.,0.,0.));
#12134=DIRECTION('',(1.,0.,0.));
#12135=DIRECTION('center_axis',(0.,0.,-1.));
#12136=DIRECTION('ref_axis',(1.,0.,0.));
#12137=DIRECTION('center_axis',(0.,0.,-1.));
#12138=DIRECTION('ref_axis',(-1.,0.,0.));
#12139=DIRECTION('',(1.,0.,0.));
#12140=DIRECTION('',(1.,0.,0.));
#12141=DIRECTION('center_axis',(0.,0.,-1.));
#12142=DIRECTION('ref_axis',(-1.,0.,0.));
#12143=DIRECTION('',(-1.,0.,0.));
#12144=DIRECTION('',(0.,-1.,0.));
#12145=DIRECTION('',(0.,-1.,0.));
#12146=DIRECTION('center_axis',(0.,1.,0.));
#12147=DIRECTION('ref_axis',(0.,0.,1.));
#12148=DIRECTION('',(0.,0.,-1.));
#12149=DIRECTION('',(-1.,0.,0.));
#12150=DIRECTION('',(0.,0.,-1.));
#12151=DIRECTION('',(-1.,0.,0.));
#12152=DIRECTION('center_axis',(1.,0.,0.));
#12153=DIRECTION('ref_axis',(0.,0.,-1.));
#12154=DIRECTION('',(0.,1.,0.));
#12155=DIRECTION('',(0.,-1.,0.));
#12156=DIRECTION('',(0.,0.,-1.));
#12157=DIRECTION('center_axis',(0.,1.,0.));
#12158=DIRECTION('ref_axis',(0.,0.,1.));
#12159=DIRECTION('',(-1.,0.,0.));
#12160=DIRECTION('',(1.,0.,0.));
#12161=DIRECTION('',(0.,0.,-1.));
#12162=DIRECTION('center_axis',(0.,0.,-1.));
#12163=DIRECTION('ref_axis',(-1.,0.,0.));
#12164=DIRECTION('center_axis',(0.,0.,-1.));
#12165=DIRECTION('ref_axis',(-1.,0.,0.));
#12166=DIRECTION('center_axis',(0.,0.,1.));
#12167=DIRECTION('ref_axis',(1.,0.,0.));
#12168=DIRECTION('',(0.,0.,-1.));
#12169=DIRECTION('center_axis',(1.,0.,0.));
#12170=DIRECTION('ref_axis',(0.,0.,-1.));
#12171=DIRECTION('',(0.,1.,0.));
#12172=DIRECTION('',(0.,-1.,0.));
#12173=DIRECTION('',(0.,0.,1.));
#12174=DIRECTION('',(0.,0.,-1.));
#12175=DIRECTION('',(0.,0.,1.));
#12176=DIRECTION('center_axis',(0.,0.,-1.));
#12177=DIRECTION('ref_axis',(-1.,0.,0.));
#12178=DIRECTION('',(0.,0.,-1.));
#12179=DIRECTION('center_axis',(0.,1.,0.));
#12180=DIRECTION('ref_axis',(0.,0.,1.));
#12181=DIRECTION('',(0.,0.,-1.));
#12182=DIRECTION('center_axis',(0.,0.,-1.));
#12183=DIRECTION('ref_axis',(-1.,0.,0.));
#12184=DIRECTION('',(0.,0.,-1.));
#12185=DIRECTION('center_axis',(-1.,0.,0.));
#12186=DIRECTION('ref_axis',(0.,0.,1.));
#12187=DIRECTION('',(0.,0.,-1.));
#12188=DIRECTION('center_axis',(0.,0.,-1.));
#12189=DIRECTION('ref_axis',(-1.,0.,0.));
#12190=DIRECTION('',(0.,0.,-1.));
#12191=DIRECTION('center_axis',(0.,1.,0.));
#12192=DIRECTION('ref_axis',(0.,0.,1.));
#12193=DIRECTION('',(0.,0.,-1.));
#12194=DIRECTION('',(1.,0.,0.));
#12195=DIRECTION('center_axis',(-1.,0.,0.));
#12196=DIRECTION('ref_axis',(0.,0.,1.));
#12197=DIRECTION('',(0.,0.,-1.));
#12198=DIRECTION('',(0.,1.,0.));
#12199=DIRECTION('center_axis',(0.,1.,0.));
#12200=DIRECTION('ref_axis',(0.,0.,1.));
#12201=DIRECTION('',(0.,0.,-1.));
#12202=DIRECTION('',(1.,0.,0.));
#12203=DIRECTION('center_axis',(0.,0.,-1.));
#12204=DIRECTION('ref_axis',(-1.,0.,0.));
#12205=DIRECTION('',(0.,0.,-1.));
#12206=DIRECTION('center_axis',(-1.,0.,0.));
#12207=DIRECTION('ref_axis',(0.,0.,1.));
#12208=DIRECTION('',(0.,0.,-1.));
#12209=DIRECTION('center_axis',(0.,0.,-1.));
#12210=DIRECTION('ref_axis',(-1.,0.,0.));
#12211=DIRECTION('',(0.,0.,-1.));
#12212=DIRECTION('center_axis',(0.,1.,0.));
#12213=DIRECTION('ref_axis',(0.,0.,1.));
#12214=DIRECTION('',(0.,0.,-1.));
#12215=DIRECTION('center_axis',(0.,0.,-1.));
#12216=DIRECTION('ref_axis',(-1.,0.,0.));
#12217=DIRECTION('',(0.,0.,-1.));
#12218=DIRECTION('center_axis',(1.,0.,0.));
#12219=DIRECTION('ref_axis',(0.,0.,-1.));
#12220=DIRECTION('',(0.,0.,-1.));
#12221=DIRECTION('',(0.,-1.,0.));
#12222=DIRECTION('',(0.,0.,-1.));
#12223=DIRECTION('',(0.,0.,-1.));
#12224=DIRECTION('',(0.,1.,0.));
#12225=DIRECTION('center_axis',(0.,0.,-1.));
#12226=DIRECTION('ref_axis',(-1.,0.,0.));
#12227=DIRECTION('center_axis',(0.,0.,-1.));
#12228=DIRECTION('ref_axis',(-1.,0.,0.));
#12229=DIRECTION('center_axis',(0.,0.,1.));
#12230=DIRECTION('ref_axis',(1.,0.,0.));
#12231=DIRECTION('center_axis',(0.,0.,-1.));
#12232=DIRECTION('ref_axis',(-1.,0.,0.));
#12233=DIRECTION('center_axis',(0.,0.,1.));
#12234=DIRECTION('ref_axis',(1.,0.,0.));
#12235=DIRECTION('',(-1.,0.,0.));
#12236=DIRECTION('center_axis',(0.,1.,0.));
#12237=DIRECTION('ref_axis',(0.,0.,1.));
#12238=DIRECTION('center_axis',(0.,0.,-1.));
#12239=DIRECTION('ref_axis',(-1.,0.,0.));
#12240=DIRECTION('',(-1.,0.,0.));
#12241=DIRECTION('center_axis',(0.,1.,0.));
#12242=DIRECTION('ref_axis',(0.,0.,1.));
#14912=CARTESIAN_POINT('',(0.,0.,0.));
#14913=CARTESIAN_POINT('Origin',(207.953766646564,-91.,12.8058966268102));
#14914=CARTESIAN_POINT('',(207.953766646564,-4.7625,6.45589662681021));
#14915=CARTESIAN_POINT('Origin',(207.953766646564,-4.7625,12.8058966268102));
#14916=CARTESIAN_POINT('',(207.953766646564,0.,6.45589662681021));
#14917=CARTESIAN_POINT('',(207.953766646564,-91.,6.45589662681021));
#14918=CARTESIAN_POINT('Origin',(207.953766646564,0.,12.8058966268102));
#14919=CARTESIAN_POINT('Origin',(207.953766646564,-91.,88.7941033731899));
#14920=CARTESIAN_POINT('',(207.953766646564,-4.7625,82.4441033731899));
#14921=CARTESIAN_POINT('Origin',(207.953766646564,-4.7625,88.7941033731899));
#14922=CARTESIAN_POINT('',(207.953766646564,0.,82.4441033731899));
#14923=CARTESIAN_POINT('',(207.953766646564,-91.,82.4441033731899));
#14924=CARTESIAN_POINT('Origin',(207.953766646564,0.,88.7941033731899));
#14925=CARTESIAN_POINT('Origin',(19.8411166279443,-91.,50.8000000000001));
#14926=CARTESIAN_POINT('',(19.8411166279443,-4.7625,44.4500000000001));
#14927=CARTESIAN_POINT('Origin',(19.8411166279443,-4.7625,50.8000000000001));
#14928=CARTESIAN_POINT('',(19.8411166279443,0.,44.4500000000001));
#14929=CARTESIAN_POINT('',(19.8411166279443,-91.,44.4500000000001));
#14930=CARTESIAN_POINT('Origin',(19.8411166279443,0.,50.8000000000001));
#14931=CARTESIAN_POINT('Origin',(225.2375,1.,101.6));
#14932=CARTESIAN_POINT('',(225.2375,1.,101.6));
#14933=CARTESIAN_POINT('',(230.,1.,101.6));
#14934=CARTESIAN_POINT('',(225.2375,1.,101.6));
#14935=CARTESIAN_POINT('',(224.2375,0.,101.6));
#14936=CARTESIAN_POINT('Origin',(224.2375,1.,101.6));
#14937=CARTESIAN_POINT('',(224.2375,-4.7625,101.6));
#14938=CARTESIAN_POINT('',(224.2375,-4.7625,101.6));
#14939=CARTESIAN_POINT('Origin',(224.2375,1.,101.6));
#14940=CARTESIAN_POINT('Origin',(224.2375,-4.7625,101.6));
#14941=CARTESIAN_POINT('',(225.2375,59.475,101.6));
#14942=CARTESIAN_POINT('',(225.2375,0.,101.6));
#14943=CARTESIAN_POINT('',(230.,59.475,101.6));
#14944=CARTESIAN_POINT('',(230.,0.,101.6));
#14945=CARTESIAN_POINT('',(230.,59.475,101.6));
#14946=CARTESIAN_POINT('Origin',(224.2375,0.,0.));
#14947=CARTESIAN_POINT('',(224.2375,0.,0.));
#14948=CARTESIAN_POINT('',(224.2375,-4.7625,0.));
#14949=CARTESIAN_POINT('',(224.2375,0.,0.));
#14950=CARTESIAN_POINT('',(225.2375,1.,0.));
#14951=CARTESIAN_POINT('Origin',(224.2375,1.,0.));
#14952=CARTESIAN_POINT('',(230.,1.,0.));
#14953=CARTESIAN_POINT('',(230.,1.,0.));
#14954=CARTESIAN_POINT('Origin',(224.2375,1.,0.));
#14955=CARTESIAN_POINT('Origin',(230.,1.,0.));
#14956=CARTESIAN_POINT('',(0.,0.,0.));
#14957=CARTESIAN_POINT('',(0.,0.,0.));
#14958=CARTESIAN_POINT('',(0.,-4.7625,0.));
#14959=CARTESIAN_POINT('',(0.,-4.7625,0.));
#14960=CARTESIAN_POINT('',(0.,-4.7625,0.));
#14961=CARTESIAN_POINT('Origin',(231.,65.2375,101.6));
#14962=CARTESIAN_POINT('',(231.,65.2375,101.6));
#14963=CARTESIAN_POINT('',(231.,60.475,101.6));
#14964=CARTESIAN_POINT('',(231.,65.2375,101.6));
#14965=CARTESIAN_POINT('Origin',(231.,59.475,101.6));
#14966=CARTESIAN_POINT('Origin',(231.,59.475,101.6));
#14967=CARTESIAN_POINT('Origin',(230.,59.475,101.6));
#14968=CARTESIAN_POINT('',(264.2375,65.2375,101.6));
#14969=CARTESIAN_POINT('',(225.2375,65.2375,101.6));
#14970=CARTESIAN_POINT('',(264.2375,60.475,101.6));
#14971=CARTESIAN_POINT('',(225.2375,60.475,101.6));
#14972=CARTESIAN_POINT('',(264.2375,60.475,101.6));
#14973=CARTESIAN_POINT('Origin',(225.2375,59.475,0.));
#14974=CARTESIAN_POINT('',(225.2375,59.475,0.));
#14975=CARTESIAN_POINT('',(230.,59.475,0.));
#14976=CARTESIAN_POINT('',(225.2375,59.475,0.));
#14977=CARTESIAN_POINT('',(231.,65.2375,0.));
#14978=CARTESIAN_POINT('Origin',(231.,59.475,0.));
#14979=CARTESIAN_POINT('',(231.,60.475,0.));
#14980=CARTESIAN_POINT('',(231.,60.475,0.));
#14981=CARTESIAN_POINT('Origin',(231.,59.475,0.));
#14982=CARTESIAN_POINT('Origin',(231.,60.475,0.));
#14983=CARTESIAN_POINT('',(225.2375,0.,0.));
#14984=CARTESIAN_POINT('',(230.,0.,0.));
#14985=CARTESIAN_POINT('Origin',(270.,59.475,101.6));
#14986=CARTESIAN_POINT('',(270.,59.475,101.6));
#14987=CARTESIAN_POINT('',(265.2375,59.475,101.6));
#14988=CARTESIAN_POINT('',(270.,59.475,101.6));
#14989=CARTESIAN_POINT('Origin',(264.2375,59.475,101.6));
#14990=CARTESIAN_POINT('Origin',(264.2375,59.475,101.6));
#14991=CARTESIAN_POINT('Origin',(264.2375,60.475,101.6));
#14992=CARTESIAN_POINT('',(270.,-3.54548993221453,101.6));
#14993=CARTESIAN_POINT('',(265.2375,-3.54548993221453,101.6));
#14994=CARTESIAN_POINT('',(356.2375,-3.54548993221453,101.6));
#14995=CARTESIAN_POINT('',(270.,65.2375,101.6));
#14996=CARTESIAN_POINT('',(265.2375,65.2375,101.6));
#14997=CARTESIAN_POINT('Origin',(264.2375,65.2375,0.));
#14998=CARTESIAN_POINT('',(264.2375,65.2375,0.));
#14999=CARTESIAN_POINT('',(264.2375,60.475,0.));
#15000=CARTESIAN_POINT('',(264.2375,65.2375,0.));
#15001=CARTESIAN_POINT('',(270.,59.475,0.));
#15002=CARTESIAN_POINT('Origin',(264.2375,59.475,0.));
#15003=CARTESIAN_POINT('',(265.2375,59.475,0.));
#15004=CARTESIAN_POINT('',(265.2375,59.475,0.));
#15005=CARTESIAN_POINT('Origin',(264.2375,59.475,0.));
#15006=CARTESIAN_POINT('Origin',(265.2375,59.475,0.));
#15007=CARTESIAN_POINT('',(225.2375,65.2375,0.));
#15008=CARTESIAN_POINT('',(225.2375,60.475,0.));
#15009=CARTESIAN_POINT('Origin',(271.,-9.525,0.));
#15010=CARTESIAN_POINT('',(270.,-3.54548993221453,0.));
#15011=CARTESIAN_POINT('',(265.2375,-3.54548993221453,0.));
#15012=CARTESIAN_POINT('',(356.2375,-3.54548993221453,0.));
#15013=CARTESIAN_POINT('',(265.2375,65.2375,0.));
#15014=CARTESIAN_POINT('',(270.,65.2375,0.));
#15015=CARTESIAN_POINT('Origin',(270.,-9.525,101.6));
#15016=CARTESIAN_POINT('',(297.294,-9.52500000000001,65.8));
#15017=CARTESIAN_POINT('',(297.294,-9.525,35.8));
#15018=CARTESIAN_POINT('',(297.294,-9.525,101.6));
#15019=CARTESIAN_POINT('',(271.,-9.52500000000001,65.8));
#15020=CARTESIAN_POINT('',(356.2375,-9.52500000000001,65.8));
#15021=CARTESIAN_POINT('',(271.,-9.525,35.8));
#15022=CARTESIAN_POINT('',(271.,-9.525,101.6));
#15023=CARTESIAN_POINT('',(356.2375,-9.525,35.8));
#15024=CARTESIAN_POINT('Origin',(297.294,-4.7625,101.6));
#15025=CARTESIAN_POINT('',(297.294,-4.7625,65.8));
#15026=CARTESIAN_POINT('',(297.294,-4.7625,65.8));
#15027=CARTESIAN_POINT('',(297.294,-4.7625,35.8));
#15028=CARTESIAN_POINT('',(297.294,-4.7625,35.8));
#15029=CARTESIAN_POINT('',(297.294,-4.7625,101.6));
#15030=CARTESIAN_POINT('Origin',(270.,-4.7625,101.6));
#15031=CARTESIAN_POINT('',(271.,-4.7625,65.8));
#15032=CARTESIAN_POINT('',(270.,-4.7625,65.8));
#15033=CARTESIAN_POINT('',(271.,-4.7625,35.8));
#15034=CARTESIAN_POINT('',(270.,-4.7625,35.8));
#15035=CARTESIAN_POINT('',(271.,-4.7625,101.6));
#15036=CARTESIAN_POINT('Origin',(271.,-3.7625,101.6));
#15037=CARTESIAN_POINT('',(270.,-3.7625,65.8));
#15038=CARTESIAN_POINT('Origin',(271.,-3.7625,65.8));
#15039=CARTESIAN_POINT('',(270.,-3.7625,35.8));
#15040=CARTESIAN_POINT('Origin',(271.,-3.7625,35.8));
#15041=CARTESIAN_POINT('',(270.,-3.7625,101.6));
#15042=CARTESIAN_POINT('Origin',(270.,65.2375,101.6));
#15043=CARTESIAN_POINT('',(270.,-3.54548993221453,65.8));
#15044=CARTESIAN_POINT('',(270.,65.2375,65.8));
#15045=CARTESIAN_POINT('',(270.,-3.54548993221453,35.8));
#15046=CARTESIAN_POINT('',(270.,65.2375,35.8));
#15047=CARTESIAN_POINT('',(270.,-3.54548993221453,101.6));
#15048=CARTESIAN_POINT('',(270.,59.475,101.6));
#15049=CARTESIAN_POINT('',(270.,-3.54548993221453,101.6));
#15050=CARTESIAN_POINT('Origin',(264.2375,59.475,101.6));
#15051=CARTESIAN_POINT('',(264.2375,65.2375,101.6));
#15052=CARTESIAN_POINT('Origin',(225.2375,65.2375,101.6));
#15053=CARTESIAN_POINT('',(231.,65.2375,101.6));
#15054=CARTESIAN_POINT('Origin',(231.,59.475,101.6));
#15055=CARTESIAN_POINT('',(225.2375,59.475,101.6));
#15056=CARTESIAN_POINT('Origin',(225.2375,0.,101.6));
#15057=CARTESIAN_POINT('',(225.2375,1.,101.6));
#15058=CARTESIAN_POINT('Origin',(224.2375,1.,101.6));
#15059=CARTESIAN_POINT('',(224.2375,0.,101.6));
#15060=CARTESIAN_POINT('Origin',(0.,0.,101.6));
#15061=CARTESIAN_POINT('',(0.,0.,101.6));
#15062=CARTESIAN_POINT('',(0.,0.,101.6));
#15063=CARTESIAN_POINT('',(0.,0.,101.6));
#15064=CARTESIAN_POINT('Origin',(0.,-4.7625,101.6));
#15065=CARTESIAN_POINT('',(0.,-4.7625,101.6));
#15066=CARTESIAN_POINT('',(0.,-4.7625,101.6));
#15067=CARTESIAN_POINT('',(0.,-4.7625,101.6));
#15068=CARTESIAN_POINT('Origin',(0.,-4.7625,101.6));
#15069=CARTESIAN_POINT('',(224.2375,-4.7625,101.6));
#15070=CARTESIAN_POINT('',(0.,-4.7625,101.6));
#15071=CARTESIAN_POINT('Origin',(224.2375,1.,101.6));
#15072=CARTESIAN_POINT('',(230.,1.,101.6));
#15073=CARTESIAN_POINT('Origin',(230.,0.,101.6));
#15074=CARTESIAN_POINT('',(230.,59.475,101.6));
#15075=CARTESIAN_POINT('Origin',(231.,59.475,101.6));
#15076=CARTESIAN_POINT('',(231.,60.475,101.6));
#15077=CARTESIAN_POINT('Origin',(225.2375,60.475,101.6));
#15078=CARTESIAN_POINT('',(264.2375,60.475,101.6));
#15079=CARTESIAN_POINT('Origin',(264.2375,59.475,101.6));
#15080=CARTESIAN_POINT('',(265.2375,59.475,101.6));
#15081=CARTESIAN_POINT('Origin',(265.2375,65.2375,101.6));
#15082=CARTESIAN_POINT('',(265.2375,-3.7625,65.8));
#15083=CARTESIAN_POINT('',(265.2375,-3.7625,35.8));
#15084=CARTESIAN_POINT('',(265.2375,-3.7625,101.6));
#15085=CARTESIAN_POINT('',(265.2375,-3.54548993221453,65.8));
#15086=CARTESIAN_POINT('',(265.2375,-9.52500000000001,65.8));
#15087=CARTESIAN_POINT('',(265.2375,-3.54548993221453,101.6));
#15088=CARTESIAN_POINT('',(265.2375,-3.54548993221453,35.8));
#15089=CARTESIAN_POINT('',(265.2375,-3.54548993221453,0.));
#15090=CARTESIAN_POINT('',(265.2375,-9.525,35.8));
#15091=CARTESIAN_POINT('Origin',(271.,-3.7625,101.6));
#15092=CARTESIAN_POINT('Origin',(271.,-3.7625,65.8));
#15093=CARTESIAN_POINT('Origin',(271.,-3.7625,35.8));
#15094=CARTESIAN_POINT('Origin',(271.,-3.7625,101.6));
#15095=CARTESIAN_POINT('Origin',(356.2375,-9.525,35.8));
#15096=CARTESIAN_POINT('',(356.2375,-3.54548993221453,35.8));
#15097=CARTESIAN_POINT('Origin',(356.2375,-3.54548993221453,0.));
#15098=CARTESIAN_POINT('Origin',(356.2375,-9.52500000000001,65.8));
#15099=CARTESIAN_POINT('',(356.2375,-3.54548993221453,65.8));
#15100=CARTESIAN_POINT('Origin',(356.2375,-3.54548993221453,101.6));
#17972=UNCERTAINTY_MEASURE_WITH_UNIT(LENGTH_MEASURE(0.01),#18007,
'DISTANCE_ACCURACY_VALUE',
'Maximum model space distance between geometric entities at asserted c
onnectivities');
#17986=UNCERTAINTY_MEASURE_WITH_UNIT(LENGTH_MEASURE(0.01),#18007,
'DISTANCE_ACCURACY_VALUE',
'Maximum model space distance between geometric entities at asserted c
onnectivities');
#17992=(
GEOMETRIC_REPRESENTATION_CONTEXT(3)
GLOBAL_UNCERTAINTY_ASSIGNED_CONTEXT((#17972))
GLOBAL_UNIT_ASSIGNED_CONTEXT((#18007,#18009,#18010))
REPRESENTATION_CONTEXT('','3D')
);
#18006=(
GEOMETRIC_REPRESENTATION_CONTEXT(3)
GLOBAL_UNCERTAINTY_ASSIGNED_CONTEXT((#17986))
GLOBAL_UNIT_ASSIGNED_CONTEXT((#18007,#18009,#18010))
REPRESENTATION_CONTEXT('','3D')
);
#18007=(
LENGTH_UNIT()
NAMED_UNIT(*)
SI_UNIT(.MILLI.,.METRE.)
);
#18009=(
NAMED_UNIT(*)
PLANE_ANGLE_UNIT()
SI_UNIT($,.RADIAN.)
);
#18010=(
NAMED_UNIT(*)
SI_UNIT($,.STERADIAN.)
SOLID_ANGLE_UNIT()
);
#18016=SHAPE_DEFINITION_REPRESENTATION(#18035,#18075);
#18035=PRODUCT_DEFINITION_SHAPE('',$,#18095);
#18075=SHAPE_REPRESENTATION('',(#10147),#17992);
#18089=PRODUCT_DEFINITION_CONTEXT('part definition',#18148,'design');
#18095=PRODUCT_DEFINITION('Mounting Strap','Mounting Strap',#18114,#18089);
#18114=PRODUCT_DEFINITION_FORMATION('',$,#18155);
#18148=APPLICATION_CONTEXT(
'Core Data for Automotive Mechanical Design Process');
#18149=PRODUCT_CONTEXT('part definition',#18148,'mechanical');
#18155=PRODUCT('Mounting Strap','Mounting Strap',$,(#18149));
#18172=PRESENTATION_STYLE_ASSIGNMENT((#18176));
#18176=SURFACE_STYLE_USAGE(.BOTH.,#18180);
#18180=SURFACE_SIDE_STYLE('',(#18184));
#18184=SURFACE_STYLE_FILL_AREA(#18188);
#18188=FILL_AREA_STYLE('Opaque(97,158,199)',(#18192));
#18192=FILL_AREA_STYLE_COLOUR('Opaque(97,158,199)',#18196);
#18196=COLOUR_RGB('Opaque(97,158,199)',0.380392156862745,0.619607843137255,
0.780392156862745);
ENDSEC;
END-ISO-10303-21;
